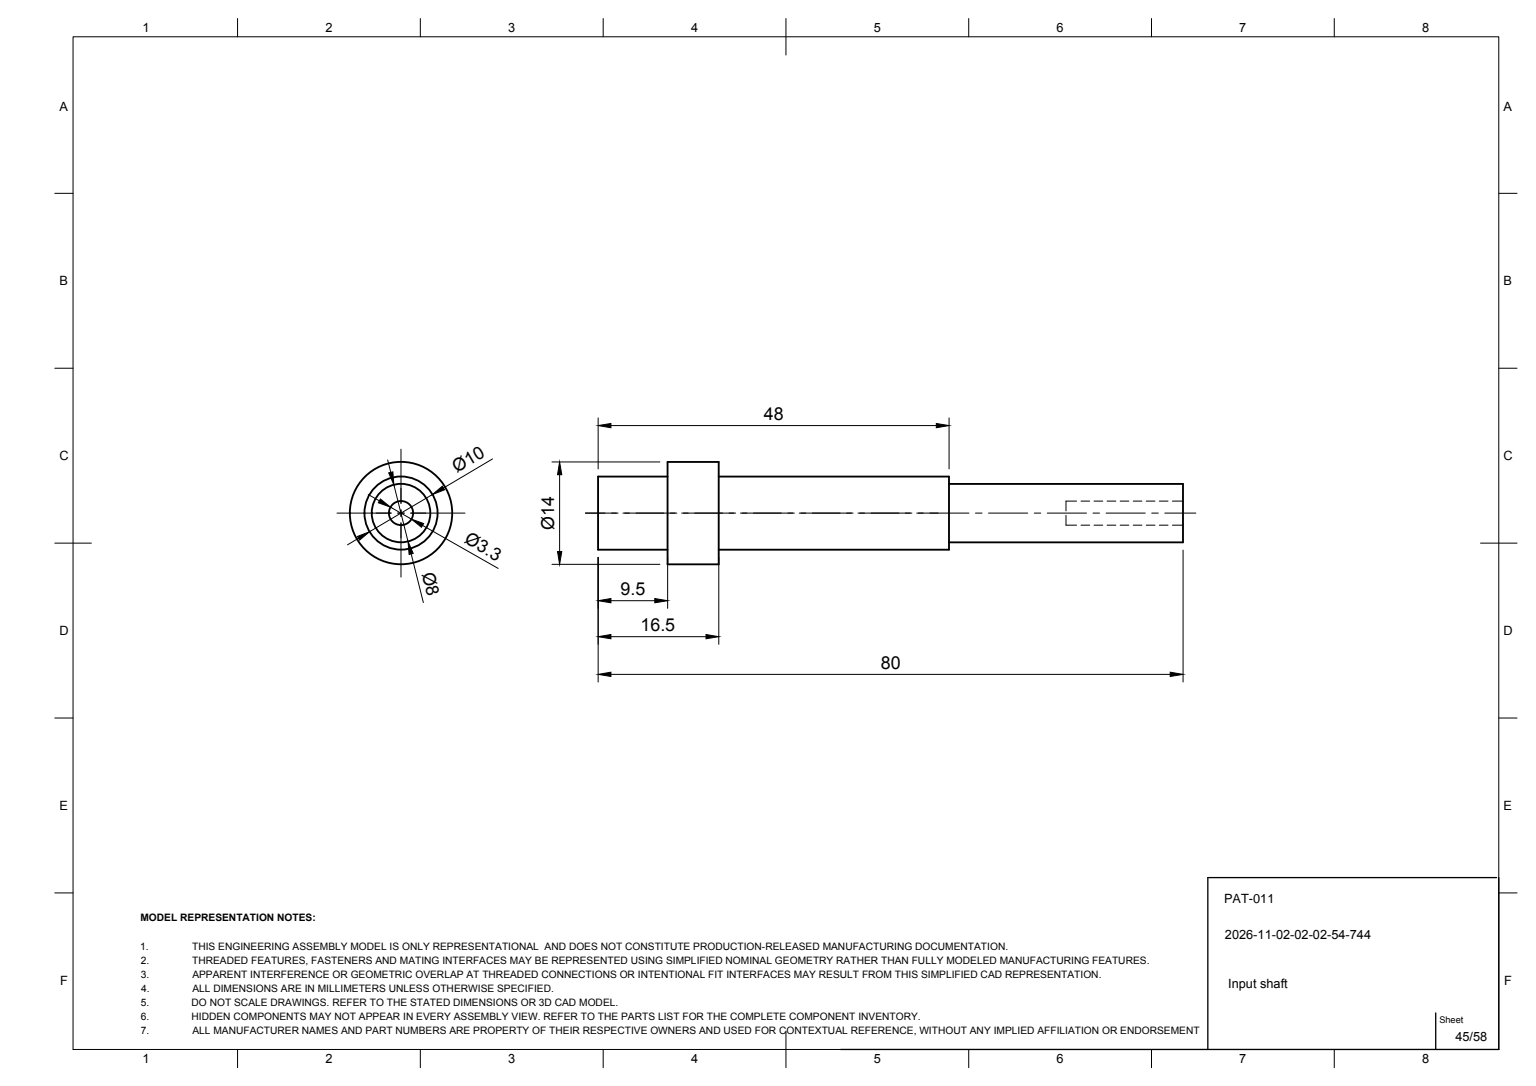
ISO-10303-21;
HEADER;
/* Generated by software containing ST-Developer
 * from STEP Tools, Inc. (www.steptools.com) 
 */

FILE_DESCRIPTION(
/* description */ ('Belt tension measurement rig'),
/* implementation_level */ '2;1');

FILE_NAME(
/* name */ 'Input shaft.step',
/* time_stamp */ '2026-10-28T03:24:44-07:00',
/* author */ (''),
/* organization */ (''),
/* preprocessor_version */ 'ST-DEVELOPER v20.2',
/* originating_system */ 'Autodesk Translation Framework v15.17.0.0',
/* authorisation */ '');

FILE_SCHEMA (('AUTOMOTIVE_DESIGN { 1 0 10303 214 3 1 1 }'));
ENDSEC;

DATA;
#10=MECHANICAL_DESIGN_GEOMETRIC_PRESENTATION_REPRESENTATION('',(#744),#23587);
#619=SHAPE_REPRESENTATION_RELATIONSHIP('SRR','None',#23869,#674);
#674=ADVANCED_BREP_SHAPE_REPRESENTATION('',(#812),#23567);
#744=STYLED_ITEM('',(#24211),#812);
#812=MANIFOLD_SOLID_BREP('Body1',#12251);
#984=FACE_BOUND('',#2661,.T.);
#985=FACE_BOUND('',#2663,.T.);
#986=FACE_BOUND('',#2668,.T.);
#987=FACE_BOUND('',#2672,.T.);
#1277=PLANE('',#13810);
#1278=PLANE('',#13811);
#1279=PLANE('',#13814);
#1280=PLANE('',#13823);
#1281=PLANE('',#13826);
#1282=PLANE('',#13827);
#1799=FACE_OUTER_BOUND('',#2658,.T.);
#1800=FACE_OUTER_BOUND('',#2659,.T.);
#1801=FACE_OUTER_BOUND('',#2660,.T.);
#1802=FACE_OUTER_BOUND('',#2662,.T.);
#1803=FACE_OUTER_BOUND('',#2664,.T.);
#1804=FACE_OUTER_BOUND('',#2665,.T.);
#1805=FACE_OUTER_BOUND('',#2666,.T.);
#1806=FACE_OUTER_BOUND('',#2667,.T.);
#1807=FACE_OUTER_BOUND('',#2669,.T.);
#1808=FACE_OUTER_BOUND('',#2670,.T.);
#1809=FACE_OUTER_BOUND('',#2671,.T.);
#2658=EDGE_LOOP('',(#9920,#9921,#9922,#9923));
#2659=EDGE_LOOP('',(#9924));
#2660=EDGE_LOOP('',(#9925));
#2661=EDGE_LOOP('',(#9926));
#2662=EDGE_LOOP('',(#9927));
#2663=EDGE_LOOP('',(#9928));
#2664=EDGE_LOOP('',(#9929,#9930,#9931,#9932));
#2665=EDGE_LOOP('',(#9933,#9934,#9935,#9936));
#2666=EDGE_LOOP('',(#9937,#9938,#9939,#9940));
#2667=EDGE_LOOP('',(#9941));
#2668=EDGE_LOOP('',(#9942));
#2669=EDGE_LOOP('',(#9943,#9944,#9945,#9946));
#2670=EDGE_LOOP('',(#9947));
#2671=EDGE_LOOP('',(#9948));
#2672=EDGE_LOOP('',(#9949));
#3493=LINE('',#21447,#4244);
#3494=LINE('',#21461,#4245);
#3495=LINE('',#21464,#4246);
#3496=LINE('',#21470,#4247);
#3497=LINE('',#21476,#4248);
#4244=VECTOR('',#16908,0.165);
#4245=VECTOR('',#16927,0.7);
#4246=VECTOR('',#16930,0.5);
#4247=VECTOR('',#16937,0.4);
#4248=VECTOR('',#16946,0.5);
#4896=CIRCLE('',#13808,0.165);
#4897=CIRCLE('',#13809,0.165);
#4898=CIRCLE('',#13812,0.7);
#4899=CIRCLE('',#13813,0.5);
#4900=CIRCLE('',#13815,0.7);
#4901=CIRCLE('',#13816,0.5);
#4902=CIRCLE('',#13819,0.5);
#4903=CIRCLE('',#13821,0.4);
#4904=CIRCLE('',#13822,0.4);
#4905=CIRCLE('',#13825,0.5);
#5911=VERTEX_POINT('',#21444);
#5912=VERTEX_POINT('',#21446);
#5913=VERTEX_POINT('',#21451);
#5914=VERTEX_POINT('',#21453);
#5915=VERTEX_POINT('',#21456);
#5916=VERTEX_POINT('',#21458);
#5917=VERTEX_POINT('',#21463);
#5918=VERTEX_POINT('',#21467);
#5919=VERTEX_POINT('',#21469);
#5920=VERTEX_POINT('',#21474);
#7319=EDGE_CURVE('',#5911,#5911,#4896,.T.);
#7320=EDGE_CURVE('',#5911,#5912,#3493,.T.);
#7321=EDGE_CURVE('',#5912,#5912,#4897,.T.);
#7322=EDGE_CURVE('',#5913,#5913,#4898,.T.);
#7323=EDGE_CURVE('',#5914,#5914,#4899,.T.);
#7324=EDGE_CURVE('',#5915,#5915,#4900,.T.);
#7325=EDGE_CURVE('',#5916,#5916,#4901,.T.);
#7326=EDGE_CURVE('',#5913,#5915,#3494,.T.);
#7327=EDGE_CURVE('',#5916,#5917,#3495,.T.);
#7328=EDGE_CURVE('',#5917,#5917,#4902,.T.);
#7329=EDGE_CURVE('',#5918,#5918,#4903,.T.);
#7330=EDGE_CURVE('',#5918,#5919,#3496,.T.);
#7331=EDGE_CURVE('',#5919,#5919,#4904,.T.);
#7332=EDGE_CURVE('',#5920,#5920,#4905,.T.);
#7333=EDGE_CURVE('',#5920,#5914,#3497,.T.);
#9920=ORIENTED_EDGE('',*,*,#7319,.F.);
#9921=ORIENTED_EDGE('',*,*,#7320,.T.);
#9922=ORIENTED_EDGE('',*,*,#7321,.T.);
#9923=ORIENTED_EDGE('',*,*,#7320,.F.);
#9924=ORIENTED_EDGE('',*,*,#7321,.F.);
#9925=ORIENTED_EDGE('',*,*,#7322,.T.);
#9926=ORIENTED_EDGE('',*,*,#7323,.F.);
#9927=ORIENTED_EDGE('',*,*,#7324,.F.);
#9928=ORIENTED_EDGE('',*,*,#7325,.F.);
#9929=ORIENTED_EDGE('',*,*,#7322,.F.);
#9930=ORIENTED_EDGE('',*,*,#7326,.T.);
#9931=ORIENTED_EDGE('',*,*,#7324,.T.);
#9932=ORIENTED_EDGE('',*,*,#7326,.F.);
#9933=ORIENTED_EDGE('',*,*,#7325,.T.);
#9934=ORIENTED_EDGE('',*,*,#7327,.T.);
#9935=ORIENTED_EDGE('',*,*,#7328,.T.);
#9936=ORIENTED_EDGE('',*,*,#7327,.F.);
#9937=ORIENTED_EDGE('',*,*,#7329,.F.);
#9938=ORIENTED_EDGE('',*,*,#7330,.T.);
#9939=ORIENTED_EDGE('',*,*,#7331,.T.);
#9940=ORIENTED_EDGE('',*,*,#7330,.F.);
#9941=ORIENTED_EDGE('',*,*,#7331,.F.);
#9942=ORIENTED_EDGE('',*,*,#7319,.T.);
#9943=ORIENTED_EDGE('',*,*,#7332,.F.);
#9944=ORIENTED_EDGE('',*,*,#7333,.T.);
#9945=ORIENTED_EDGE('',*,*,#7323,.T.);
#9946=ORIENTED_EDGE('',*,*,#7333,.F.);
#9947=ORIENTED_EDGE('',*,*,#7332,.T.);
#9948=ORIENTED_EDGE('',*,*,#7328,.F.);
#9949=ORIENTED_EDGE('',*,*,#7329,.T.);
#11317=CYLINDRICAL_SURFACE('',#13807,0.165);
#11318=CYLINDRICAL_SURFACE('',#13817,0.7);
#11319=CYLINDRICAL_SURFACE('',#13818,0.5);
#11320=CYLINDRICAL_SURFACE('',#13820,0.4);
#11321=CYLINDRICAL_SURFACE('',#13824,0.5);
#11940=ADVANCED_FACE('',(#1799),#11317,.F.);
#11941=ADVANCED_FACE('',(#1800),#1277,.F.);
#11942=ADVANCED_FACE('',(#1801,#984),#1278,.T.);
#11943=ADVANCED_FACE('',(#1802,#985),#1279,.F.);
#11944=ADVANCED_FACE('',(#1803),#11318,.T.);
#11945=ADVANCED_FACE('',(#1804),#11319,.T.);
#11946=ADVANCED_FACE('',(#1805),#11320,.T.);
#11947=ADVANCED_FACE('',(#1806,#986),#1280,.F.);
#11948=ADVANCED_FACE('',(#1807),#11321,.T.);
#11949=ADVANCED_FACE('',(#1808),#1281,.T.);
#11950=ADVANCED_FACE('',(#1809,#987),#1282,.F.);
#12251=CLOSED_SHELL('',(#11940,#11941,#11942,#11943,#11944,#11945,#11946,
#11947,#11948,#11949,#11950));
#13806=AXIS2_PLACEMENT_3D('',#21442,#16902,#16903);
#13807=AXIS2_PLACEMENT_3D('',#21443,#16904,#16905);
#13808=AXIS2_PLACEMENT_3D('',#21445,#16906,#16907);
#13809=AXIS2_PLACEMENT_3D('',#21448,#16909,#16910);
#13810=AXIS2_PLACEMENT_3D('',#21449,#16911,#16912);
#13811=AXIS2_PLACEMENT_3D('',#21450,#16913,#16914);
#13812=AXIS2_PLACEMENT_3D('',#21452,#16915,#16916);
#13813=AXIS2_PLACEMENT_3D('',#21454,#16917,#16918);
#13814=AXIS2_PLACEMENT_3D('',#21455,#16919,#16920);
#13815=AXIS2_PLACEMENT_3D('',#21457,#16921,#16922);
#13816=AXIS2_PLACEMENT_3D('',#21459,#16923,#16924);
#13817=AXIS2_PLACEMENT_3D('',#21460,#16925,#16926);
#13818=AXIS2_PLACEMENT_3D('',#21462,#16928,#16929);
#13819=AXIS2_PLACEMENT_3D('',#21465,#16931,#16932);
#13820=AXIS2_PLACEMENT_3D('',#21466,#16933,#16934);
#13821=AXIS2_PLACEMENT_3D('',#21468,#16935,#16936);
#13822=AXIS2_PLACEMENT_3D('',#21471,#16938,#16939);
#13823=AXIS2_PLACEMENT_3D('',#21472,#16940,#16941);
#13824=AXIS2_PLACEMENT_3D('',#21473,#16942,#16943);
#13825=AXIS2_PLACEMENT_3D('',#21475,#16944,#16945);
#13826=AXIS2_PLACEMENT_3D('',#21477,#16947,#16948);
#13827=AXIS2_PLACEMENT_3D('',#21478,#16949,#16950);
#16902=DIRECTION('axis',(0.,0.,1.));
#16903=DIRECTION('refdir',(1.,0.,0.));
#16904=DIRECTION('center_axis',(0.,1.,0.));
#16905=DIRECTION('ref_axis',(1.,0.,0.));
#16906=DIRECTION('center_axis',(0.,1.,0.));
#16907=DIRECTION('ref_axis',(1.,0.,0.));
#16908=DIRECTION('',(0.,1.,0.));
#16909=DIRECTION('center_axis',(0.,1.,0.));
#16910=DIRECTION('ref_axis',(1.,0.,0.));
#16911=DIRECTION('center_axis',(0.,1.,0.));
#16912=DIRECTION('ref_axis',(1.,0.,0.));
#16913=DIRECTION('center_axis',(0.,1.,0.));
#16914=DIRECTION('ref_axis',(1.,0.,0.));
#16915=DIRECTION('center_axis',(0.,1.,0.));
#16916=DIRECTION('ref_axis',(1.,0.,0.));
#16917=DIRECTION('center_axis',(0.,1.,0.));
#16918=DIRECTION('ref_axis',(1.,0.,0.));
#16919=DIRECTION('center_axis',(0.,1.,0.));
#16920=DIRECTION('ref_axis',(1.,0.,0.));
#16921=DIRECTION('center_axis',(0.,1.,0.));
#16922=DIRECTION('ref_axis',(1.,0.,0.));
#16923=DIRECTION('center_axis',(0.,-1.,0.));
#16924=DIRECTION('ref_axis',(1.,0.,0.));
#16925=DIRECTION('center_axis',(0.,1.,0.));
#16926=DIRECTION('ref_axis',(1.,0.,0.));
#16927=DIRECTION('',(0.,-1.,0.));
#16928=DIRECTION('center_axis',(0.,1.,0.));
#16929=DIRECTION('ref_axis',(1.,0.,0.));
#16930=DIRECTION('',(0.,-1.,0.));
#16931=DIRECTION('center_axis',(0.,1.,0.));
#16932=DIRECTION('ref_axis',(1.,0.,0.));
#16933=DIRECTION('center_axis',(0.,1.,0.));
#16934=DIRECTION('ref_axis',(1.,0.,0.));
#16935=DIRECTION('center_axis',(0.,1.,0.));
#16936=DIRECTION('ref_axis',(1.,0.,0.));
#16937=DIRECTION('',(0.,-1.,0.));
#16938=DIRECTION('center_axis',(0.,1.,0.));
#16939=DIRECTION('ref_axis',(1.,0.,0.));
#16940=DIRECTION('center_axis',(0.,1.,0.));
#16941=DIRECTION('ref_axis',(1.,0.,0.));
#16942=DIRECTION('center_axis',(0.,1.,0.));
#16943=DIRECTION('ref_axis',(1.,0.,0.));
#16944=DIRECTION('center_axis',(0.,1.,0.));
#16945=DIRECTION('ref_axis',(1.,0.,0.));
#16946=DIRECTION('',(0.,-1.,0.));
#16947=DIRECTION('center_axis',(0.,1.,0.));
#16948=DIRECTION('ref_axis',(1.,0.,0.));
#16949=DIRECTION('center_axis',(0.,1.,0.));
#16950=DIRECTION('ref_axis',(1.,0.,0.));
#21442=CARTESIAN_POINT('',(0.,0.,0.));
#21443=CARTESIAN_POINT('Origin',(0.,-5.1,7.));
#21444=CARTESIAN_POINT('',(-0.165,-5.,7.));
#21445=CARTESIAN_POINT('Origin',(0.,-5.,7.));
#21446=CARTESIAN_POINT('',(-0.165,-3.4,7.));
#21447=CARTESIAN_POINT('',(-0.165,-5.1,7.));
#21448=CARTESIAN_POINT('Origin',(0.,-3.4,7.));
#21449=CARTESIAN_POINT('Origin',(0.,-3.4,7.));
#21450=CARTESIAN_POINT('Origin',(0.,2.05,7.));
#21451=CARTESIAN_POINT('',(-0.7,2.05,7.));
#21452=CARTESIAN_POINT('Origin',(0.,2.05,7.));
#21453=CARTESIAN_POINT('',(-0.5,2.05,7.));
#21454=CARTESIAN_POINT('Origin',(0.,2.05,7.));
#21455=CARTESIAN_POINT('Origin',(0.,1.35,7.));
#21456=CARTESIAN_POINT('',(-0.7,1.35,7.));
#21457=CARTESIAN_POINT('Origin',(0.,1.35,7.));
#21458=CARTESIAN_POINT('',(-0.5,1.35,7.));
#21459=CARTESIAN_POINT('Origin',(0.,1.35,7.));
#21460=CARTESIAN_POINT('Origin',(0.,1.35,7.));
#21461=CARTESIAN_POINT('',(-0.7,1.35,7.));
#21462=CARTESIAN_POINT('Origin',(0.,-1.8,7.));
#21463=CARTESIAN_POINT('',(-0.5,-1.8,7.));
#21464=CARTESIAN_POINT('',(-0.5,-1.8,7.));
#21465=CARTESIAN_POINT('Origin',(0.,-1.8,7.));
#21466=CARTESIAN_POINT('Origin',(0.,-5.,7.));
#21467=CARTESIAN_POINT('',(-0.4,-1.8,7.));
#21468=CARTESIAN_POINT('Origin',(0.,-1.8,7.));
#21469=CARTESIAN_POINT('',(-0.4,-5.,7.));
#21470=CARTESIAN_POINT('',(-0.4,-5.,7.));
#21471=CARTESIAN_POINT('Origin',(0.,-5.,7.));
#21472=CARTESIAN_POINT('Origin',(0.,-5.,7.));
#21473=CARTESIAN_POINT('Origin',(0.,-1.8,7.));
#21474=CARTESIAN_POINT('',(-0.5,3.,7.));
#21475=CARTESIAN_POINT('Origin',(0.,3.,7.));
#21476=CARTESIAN_POINT('',(-0.5,-1.8,7.));
#21477=CARTESIAN_POINT('Origin',(0.,3.,7.));
#21478=CARTESIAN_POINT('Origin',(0.,-1.8,7.));
#23502=UNCERTAINTY_MEASURE_WITH_UNIT(LENGTH_MEASURE(0.001),#23588,
'DISTANCE_ACCURACY_VALUE',
'Maximum model space distance between geometric entities at asserted c
onnectivities');
#23522=UNCERTAINTY_MEASURE_WITH_UNIT(LENGTH_MEASURE(0.001),#23588,
'DISTANCE_ACCURACY_VALUE',
'Maximum model space distance between geometric entities at asserted c
onnectivities');
#23567=(
GEOMETRIC_REPRESENTATION_CONTEXT(3)
GLOBAL_UNCERTAINTY_ASSIGNED_CONTEXT((#23502))
GLOBAL_UNIT_ASSIGNED_CONTEXT((#23588,#23590,#23591))
REPRESENTATION_CONTEXT('','3D')
);
#23587=(
GEOMETRIC_REPRESENTATION_CONTEXT(3)
GLOBAL_UNCERTAINTY_ASSIGNED_CONTEXT((#23522))
GLOBAL_UNIT_ASSIGNED_CONTEXT((#23588,#23590,#23591))
REPRESENTATION_CONTEXT('','3D')
);
#23588=(
LENGTH_UNIT()
NAMED_UNIT(*)
SI_UNIT(.CENTI.,.METRE.)
);
#23590=(
NAMED_UNIT(*)
PLANE_ANGLE_UNIT()
SI_UNIT($,.RADIAN.)
);
#23591=(
NAMED_UNIT(*)
SI_UNIT($,.STERADIAN.)
SOLID_ANGLE_UNIT()
);
#23636=SHAPE_DEFINITION_REPRESENTATION(#23713,#23869);
#23713=PRODUCT_DEFINITION_SHAPE('',$,#23934);
#23869=SHAPE_REPRESENTATION('',(#13806),#23567);
#23889=PRODUCT_DEFINITION_CONTEXT('part definition',#24083,'design');
#23934=PRODUCT_DEFINITION('Input shaft','Input shaft',#23998,#23889);
#23998=PRODUCT_DEFINITION_FORMATION('',$,#24129);
#24083=APPLICATION_CONTEXT(
'Core Data for Automotive Mechanical Design Process');
#24084=PRODUCT_CONTEXT('part definition',#24083,'mechanical');
#24129=PRODUCT('Input shaft','Input shaft','Input shaft',(#24084));
#24205=COLOUR_RGB('Grey',0.48,0.52,0.57);
#24206=FILL_AREA_STYLE_COLOUR('',#24205);
#24207=FILL_AREA_STYLE('',(#24206));
#24208=SURFACE_STYLE_FILL_AREA(#24207);
#24209=SURFACE_SIDE_STYLE('',(#24208));
#24210=SURFACE_STYLE_USAGE(.BOTH.,#24209);
#24211=PRESENTATION_STYLE_ASSIGNMENT((#24210));
ENDSEC;
END-ISO-10303-21;
